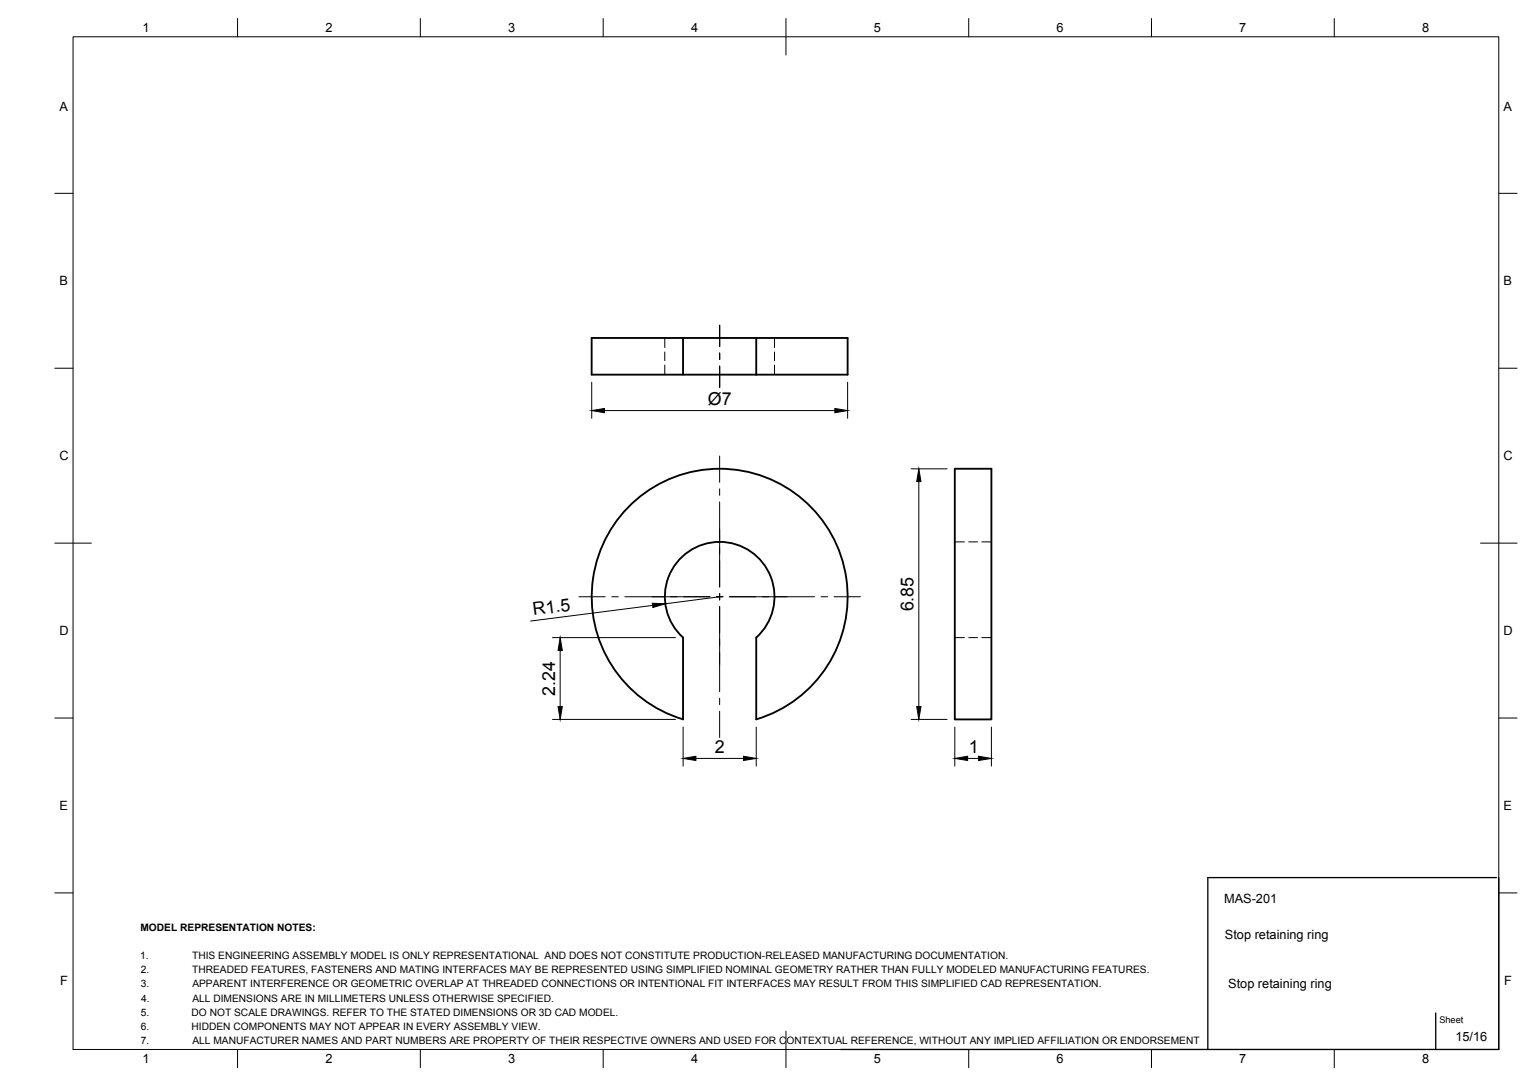
ISO-10303-21;
HEADER;
/* Generated by software containing ST-Developer
 * from STEP Tools, Inc. (www.steptools.com) 
 */

FILE_DESCRIPTION(
/* description */ ('Independent manual two-gate roller-track escapement for nominal30mm d
iameter20mm wide feed rollers. Opposed gates are driven by native capt
ured pin-slot loops with positive curved-slot travel stops at\X\B116de
g. Repeated gate/pin/washer/clip instances, adapted native common bear
ing families, full retaining lips and rotating polymer grip. External 
workpieces, gravity feeder/incline and mount anchors outside assembly.
 No powered-feed compatibility, impact, capacity, safety, force, wear 
or life rating.'),
/* implementation_level */ '2;1');

FILE_NAME(
/* name */ 'Stop retaining ring.step',
/* time_stamp */ '2026-11-08T18:43:23-08:00',
/* author */ (''),
/* organization */ (''),
/* preprocessor_version */ 'ST-DEVELOPER v20.2',
/* originating_system */ 'Autodesk Translation Framework v15.17.0.0',
/* authorisation */ '');

FILE_SCHEMA (('AUTOMOTIVE_DESIGN { 1 0 10303 214 3 1 1 }'));
ENDSEC;

DATA;
#10=MECHANICAL_DESIGN_GEOMETRIC_PRESENTATION_REPRESENTATION('',(#470),#19863);
#432=SHAPE_REPRESENTATION_RELATIONSHIP('SRR','None',#19950,#451);
#451=ADVANCED_BREP_SHAPE_REPRESENTATION('',(#489),#19859);
#470=STYLED_ITEM('',(#20044),#489);
#489=MANIFOLD_SOLID_BREP('Body1',#6439);
#866=LINE('',#16006,#1331);
#867=LINE('',#16008,#1332);
#868=LINE('',#16010,#1333);
#869=LINE('',#16011,#1334);
#870=LINE('',#16015,#1335);
#871=LINE('',#16017,#1336);
#872=LINE('',#16019,#1337);
#873=LINE('',#16020,#1338);
#1331=VECTOR('',#8374,10.);
#1332=VECTOR('',#8375,10.);
#1333=VECTOR('',#8376,10.);
#1334=VECTOR('',#8377,10.);
#1335=VECTOR('',#8380,10.);
#1336=VECTOR('',#8381,10.);
#1337=VECTOR('',#8382,10.);
#1338=VECTOR('',#8383,10.);
#1564=CYLINDRICAL_SURFACE('',#7062,1.5);
#1565=CYLINDRICAL_SURFACE('',#7064,3.5);
#1960=FACE_OUTER_BOUND('',#2382,.T.);
#1961=FACE_OUTER_BOUND('',#2383,.T.);
#1962=FACE_OUTER_BOUND('',#2384,.T.);
#1963=FACE_OUTER_BOUND('',#2385,.T.);
#1964=FACE_OUTER_BOUND('',#2386,.T.);
#1965=FACE_OUTER_BOUND('',#2387,.T.);
#2382=EDGE_LOOP('',(#5481,#5482,#5483,#5484));
#2383=EDGE_LOOP('',(#5485,#5486,#5487,#5488));
#2384=EDGE_LOOP('',(#5489,#5490,#5491,#5492));
#2385=EDGE_LOOP('',(#5493,#5494,#5495,#5496));
#2386=EDGE_LOOP('',(#5497,#5498,#5499,#5500));
#2387=EDGE_LOOP('',(#5501,#5502,#5503,#5504));
#2594=CIRCLE('',#7060,3.5);
#2595=CIRCLE('',#7061,1.5);
#2596=CIRCLE('',#7063,1.5);
#2597=CIRCLE('',#7065,3.5);
#3072=VERTEX_POINT('',#16004);
#3073=VERTEX_POINT('',#16005);
#3074=VERTEX_POINT('',#16007);
#3075=VERTEX_POINT('',#16009);
#3076=VERTEX_POINT('',#16013);
#3077=VERTEX_POINT('',#16014);
#3078=VERTEX_POINT('',#16016);
#3079=VERTEX_POINT('',#16018);
#3899=EDGE_CURVE('',#3072,#3073,#866,.T.);
#3900=EDGE_CURVE('',#3074,#3072,#867,.T.);
#3901=EDGE_CURVE('',#3075,#3074,#868,.T.);
#3902=EDGE_CURVE('',#3073,#3075,#869,.T.);
#3903=EDGE_CURVE('',#3076,#3077,#870,.T.);
#3904=EDGE_CURVE('',#3078,#3076,#871,.T.);
#3905=EDGE_CURVE('',#3079,#3078,#872,.T.);
#3906=EDGE_CURVE('',#3077,#3079,#873,.T.);
#3907=EDGE_CURVE('',#3074,#3079,#2594,.T.);
#3908=EDGE_CURVE('',#3077,#3072,#2595,.T.);
#3909=EDGE_CURVE('',#3076,#3073,#2596,.T.);
#3910=EDGE_CURVE('',#3075,#3078,#2597,.T.);
#5481=ORIENTED_EDGE('',*,*,#3899,.F.);
#5482=ORIENTED_EDGE('',*,*,#3900,.F.);
#5483=ORIENTED_EDGE('',*,*,#3901,.F.);
#5484=ORIENTED_EDGE('',*,*,#3902,.F.);
#5485=ORIENTED_EDGE('',*,*,#3903,.F.);
#5486=ORIENTED_EDGE('',*,*,#3904,.F.);
#5487=ORIENTED_EDGE('',*,*,#3905,.F.);
#5488=ORIENTED_EDGE('',*,*,#3906,.F.);
#5489=ORIENTED_EDGE('',*,*,#3906,.T.);
#5490=ORIENTED_EDGE('',*,*,#3907,.F.);
#5491=ORIENTED_EDGE('',*,*,#3900,.T.);
#5492=ORIENTED_EDGE('',*,*,#3908,.F.);
#5493=ORIENTED_EDGE('',*,*,#3903,.T.);
#5494=ORIENTED_EDGE('',*,*,#3908,.T.);
#5495=ORIENTED_EDGE('',*,*,#3899,.T.);
#5496=ORIENTED_EDGE('',*,*,#3909,.F.);
#5497=ORIENTED_EDGE('',*,*,#3905,.T.);
#5498=ORIENTED_EDGE('',*,*,#3910,.F.);
#5499=ORIENTED_EDGE('',*,*,#3901,.T.);
#5500=ORIENTED_EDGE('',*,*,#3907,.T.);
#5501=ORIENTED_EDGE('',*,*,#3904,.T.);
#5502=ORIENTED_EDGE('',*,*,#3909,.T.);
#5503=ORIENTED_EDGE('',*,*,#3902,.T.);
#5504=ORIENTED_EDGE('',*,*,#3910,.T.);
#6039=PLANE('',#7057);
#6040=PLANE('',#7058);
#6041=PLANE('',#7059);
#6042=PLANE('',#7066);
#6339=ADVANCED_FACE('',(#1960),#6039,.F.);
#6340=ADVANCED_FACE('',(#1961),#6040,.F.);
#6341=ADVANCED_FACE('',(#1962),#6041,.F.);
#6342=ADVANCED_FACE('',(#1963),#1564,.F.);
#6343=ADVANCED_FACE('',(#1964),#1565,.T.);
#6344=ADVANCED_FACE('',(#1965),#6042,.T.);
#6439=CLOSED_SHELL('',(#6339,#6340,#6341,#6342,#6343,#6344));
#7056=AXIS2_PLACEMENT_3D('',#16002,#8370,#8371);
#7057=AXIS2_PLACEMENT_3D('',#16003,#8372,#8373);
#7058=AXIS2_PLACEMENT_3D('',#16012,#8378,#8379);
#7059=AXIS2_PLACEMENT_3D('',#16021,#8384,#8385);
#7060=AXIS2_PLACEMENT_3D('',#16022,#8386,#8387);
#7061=AXIS2_PLACEMENT_3D('',#16023,#8388,#8389);
#7062=AXIS2_PLACEMENT_3D('',#16024,#8390,#8391);
#7063=AXIS2_PLACEMENT_3D('',#16025,#8392,#8393);
#7064=AXIS2_PLACEMENT_3D('',#16026,#8394,#8395);
#7065=AXIS2_PLACEMENT_3D('',#16027,#8396,#8397);
#7066=AXIS2_PLACEMENT_3D('',#16028,#8398,#8399);
#8370=DIRECTION('axis',(0.,0.,1.));
#8371=DIRECTION('refdir',(1.,0.,0.));
#8372=DIRECTION('center_axis',(-1.,0.,0.));
#8373=DIRECTION('ref_axis',(0.,1.,0.));
#8374=DIRECTION('',(0.,0.,1.));
#8375=DIRECTION('',(0.,-1.,0.));
#8376=DIRECTION('',(0.,0.,-1.));
#8377=DIRECTION('',(0.,1.,0.));
#8378=DIRECTION('center_axis',(1.,0.,0.));
#8379=DIRECTION('ref_axis',(0.,-1.,0.));
#8380=DIRECTION('',(0.,0.,-1.));
#8381=DIRECTION('',(0.,-1.,0.));
#8382=DIRECTION('',(0.,0.,1.));
#8383=DIRECTION('',(0.,1.,0.));
#8384=DIRECTION('center_axis',(0.,0.,1.));
#8385=DIRECTION('ref_axis',(1.,0.,0.));
#8386=DIRECTION('center_axis',(0.,0.,1.));
#8387=DIRECTION('ref_axis',(1.,0.,0.));
#8388=DIRECTION('center_axis',(0.,0.,-1.));
#8389=DIRECTION('ref_axis',(1.,0.,0.));
#8390=DIRECTION('center_axis',(0.,0.,1.));
#8391=DIRECTION('ref_axis',(6.12323399573677E-17,-1.,0.));
#8392=DIRECTION('center_axis',(0.,0.,-1.));
#8393=DIRECTION('ref_axis',(1.,0.,0.));
#8394=DIRECTION('center_axis',(0.,0.,1.));
#8395=DIRECTION('ref_axis',(6.12323399573677E-17,-1.,0.));
#8396=DIRECTION('center_axis',(0.,0.,1.));
#8397=DIRECTION('ref_axis',(1.,0.,0.));
#8398=DIRECTION('center_axis',(0.,0.,1.));
#8399=DIRECTION('ref_axis',(1.,0.,0.));
#16002=CARTESIAN_POINT('',(0.,0.,0.));
#16003=CARTESIAN_POINT('Origin',(-1.,0.,1.));
#16004=CARTESIAN_POINT('',(-1.,1.11803398874989,0.));
#16005=CARTESIAN_POINT('',(-1.,1.11803398874989,1.));
#16006=CARTESIAN_POINT('',(-1.,1.11803398874989,0.));
#16007=CARTESIAN_POINT('',(-1.,3.35410196624968,0.));
#16008=CARTESIAN_POINT('',(-1.,0.,0.));
#16009=CARTESIAN_POINT('',(-1.,3.35410196624968,1.));
#16010=CARTESIAN_POINT('',(-1.,3.35410196624968,0.));
#16011=CARTESIAN_POINT('',(-1.,0.,1.));
#16012=CARTESIAN_POINT('Origin',(1.,7.,1.));
#16013=CARTESIAN_POINT('',(1.,1.11803398874989,1.));
#16014=CARTESIAN_POINT('',(1.,1.11803398874989,0.));
#16015=CARTESIAN_POINT('',(1.,1.11803398874989,0.));
#16016=CARTESIAN_POINT('',(1.,3.35410196624968,1.));
#16017=CARTESIAN_POINT('',(1.,3.5,1.));
#16018=CARTESIAN_POINT('',(1.,3.35410196624968,0.));
#16019=CARTESIAN_POINT('',(1.,3.35410196624968,0.));
#16020=CARTESIAN_POINT('',(1.,3.5,0.));
#16021=CARTESIAN_POINT('Origin',(0.,0.,0.));
#16022=CARTESIAN_POINT('Origin',(0.,0.,0.));
#16023=CARTESIAN_POINT('Origin',(0.,0.,0.));
#16024=CARTESIAN_POINT('Origin',(0.,0.,0.));
#16025=CARTESIAN_POINT('Origin',(0.,0.,1.));
#16026=CARTESIAN_POINT('Origin',(0.,0.,0.));
#16027=CARTESIAN_POINT('Origin',(0.,0.,1.));
#16028=CARTESIAN_POINT('Origin',(0.,0.,1.));
#19838=UNCERTAINTY_MEASURE_WITH_UNIT(LENGTH_MEASURE(0.01),#19864,
'DISTANCE_ACCURACY_VALUE',
'Maximum model space distance between geometric entities at asserted c
onnectivities');
#19842=UNCERTAINTY_MEASURE_WITH_UNIT(LENGTH_MEASURE(0.01),#19864,
'DISTANCE_ACCURACY_VALUE',
'Maximum model space distance between geometric entities at asserted c
onnectivities');
#19859=(
GEOMETRIC_REPRESENTATION_CONTEXT(3)
GLOBAL_UNCERTAINTY_ASSIGNED_CONTEXT((#19838))
GLOBAL_UNIT_ASSIGNED_CONTEXT((#19864,#19866,#19867))
REPRESENTATION_CONTEXT('','3D')
);
#19863=(
GEOMETRIC_REPRESENTATION_CONTEXT(3)
GLOBAL_UNCERTAINTY_ASSIGNED_CONTEXT((#19842))
GLOBAL_UNIT_ASSIGNED_CONTEXT((#19864,#19866,#19867))
REPRESENTATION_CONTEXT('','3D')
);
#19864=(
LENGTH_UNIT()
NAMED_UNIT(*)
SI_UNIT(.MILLI.,.METRE.)
);
#19866=(
NAMED_UNIT(*)
PLANE_ANGLE_UNIT()
SI_UNIT($,.RADIAN.)
);
#19867=(
NAMED_UNIT(*)
SI_UNIT($,.STERADIAN.)
SOLID_ANGLE_UNIT()
);
#19884=SHAPE_DEFINITION_REPRESENTATION(#19904,#19950);
#19904=PRODUCT_DEFINITION_SHAPE('',$,#19971);
#19950=SHAPE_REPRESENTATION('',(#7056),#19859);
#19954=PRODUCT_DEFINITION_CONTEXT('part definition',#20016,'design');
#19971=PRODUCT_DEFINITION('Stop retaining ring','Stop retaining ring',#19991,
#19954);
#19991=PRODUCT_DEFINITION_FORMATION('',$,#20034);
#20016=APPLICATION_CONTEXT(
'Core Data for Automotive Mechanical Design Process');
#20017=PRODUCT_CONTEXT('part definition',#20016,'mechanical');
#20034=PRODUCT('Stop retaining ring','Stop retaining ring',$,(#20017));
#20044=PRESENTATION_STYLE_ASSIGNMENT((#20051));
#20051=SURFACE_STYLE_USAGE(.BOTH.,#20058);
#20058=SURFACE_SIDE_STYLE('',(#20065));
#20065=SURFACE_STYLE_FILL_AREA(#20072);
#20072=FILL_AREA_STYLE('Dark gray',(#20079));
#20079=FILL_AREA_STYLE_COLOUR('Dark gray',#20086);
#20086=COLOUR_RGB('Dark gray',0.250980392156863,0.282352941176471,0.32156862745098);
ENDSEC;
END-ISO-10303-21;
